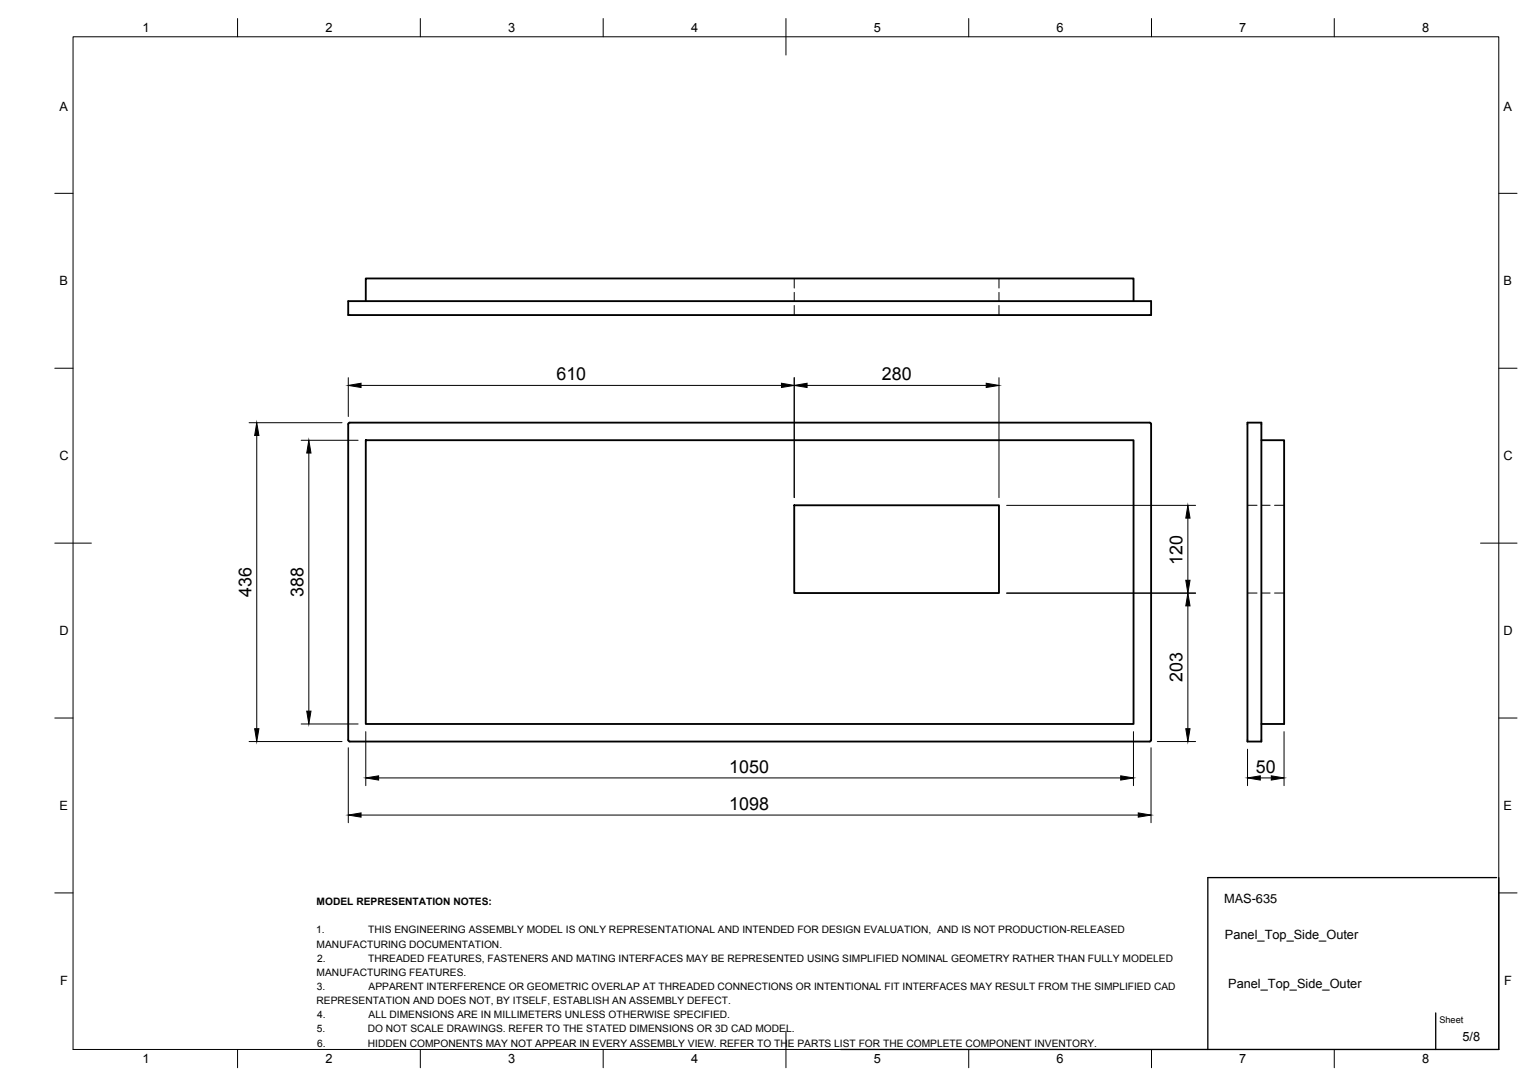
ISO-10303-21;
HEADER;
FILE_DESCRIPTION((''),'2;1');
FILE_NAME('Panel_Top_Side_Outer.step','2026-10-09T12:34:24-07:00',(''),(''),'','','');
FILE_SCHEMA (('AUTOMOTIVE_DESIGN { 1 0 10303 214 3 1 1 }'));
ENDSEC;
DATA;
#10=MECHANICAL_DESIGN_GEOMETRIC_PRESENTATION_REPRESENTATION('',(#61),#3759);
#49=SHAPE_REPRESENTATION_RELATIONSHIP('SRR','None',#3790,#55) ;
#55=ADVANCED_BREP_SHAPE_REPRESENTATION('',(#67),#3755) ;
#61=STYLED_ITEM('',(#3827),#67) ;
#67=MANIFOLD_SOLID_BREP('Body1',#2265) ;
#79=CYLINDRICAL_SURFACE('',#2421,0.2) ;
#80=CYLINDRICAL_SURFACE('',#2422,0.2) ;
#81=CYLINDRICAL_SURFACE('',#2423,0.2) ;
#82=CYLINDRICAL_SURFACE('',#2424,0.2) ;
#103=CIRCLE('',#2412,0.2) ;
#104=CIRCLE('',#2413,0.2) ;
#105=CIRCLE('',#2414,0.2) ;
#106=CIRCLE('',#2415,0.2) ;
#107=CIRCLE('',#2417,0.2) ;
#108=CIRCLE('',#2418,0.2) ;
#109=CIRCLE('',#2419,0.2) ;
#110=CIRCLE('',#2420,0.2) ;
#129=FACE_BOUND('',#322,.T.) ;
#130=FACE_BOUND('',#328,.T.) ;
#131=FACE_BOUND('',#330,.T.) ;
#187=FACE_OUTER_BOUND('',#317,.T.) ;
#188=FACE_OUTER_BOUND('',#318,.T.) ;
#189=FACE_OUTER_BOUND('',#319,.T.) ;
#190=FACE_OUTER_BOUND('',#320,.T.) ;
#191=FACE_OUTER_BOUND('',#321,.T.) ;
#192=FACE_OUTER_BOUND('',#323,.T.) ;
#193=FACE_OUTER_BOUND('',#324,.T.) ;
#194=FACE_OUTER_BOUND('',#325,.T.) ;
#195=FACE_OUTER_BOUND('',#326,.T.) ;
#196=FACE_OUTER_BOUND('',#327,.T.) ;
#197=FACE_OUTER_BOUND('',#329,.T.) ;
#198=FACE_OUTER_BOUND('',#331,.T.) ;
#199=FACE_OUTER_BOUND('',#332,.T.) ;
#200=FACE_OUTER_BOUND('',#333,.T.) ;
#201=FACE_OUTER_BOUND('',#334,.T.) ;
#202=FACE_OUTER_BOUND('',#335,.T.) ;
#203=FACE_OUTER_BOUND('',#336,.T.) ;
#204=FACE_OUTER_BOUND('',#337,.T.) ;
#205=FACE_OUTER_BOUND('',#338,.T.) ;
#317=EDGE_LOOP('',(#1679,#1680,#1681,#1682)) ;
#318=EDGE_LOOP('',(#1683,#1684,#1685,#1686)) ;
#319=EDGE_LOOP('',(#1687,#1688,#1689,#1690)) ;
#320=EDGE_LOOP('',(#1691,#1692,#1693,#1694)) ;
#321=EDGE_LOOP('',(#1695,#1696,#1697,#1698)) ;
#322=EDGE_LOOP('',(#1699,#1700,#1701,#1702)) ;
#323=EDGE_LOOP('',(#1703,#1704,#1705,#1706)) ;
#324=EDGE_LOOP('',(#1707,#1708,#1709,#1710)) ;
#325=EDGE_LOOP('',(#1711,#1712,#1713,#1714)) ;
#326=EDGE_LOOP('',(#1715,#1716,#1717,#1718)) ;
#327=EDGE_LOOP('',(#1719,#1720,#1721,#1722,#1723,#1724,#1725,#1726)) ;
#328=EDGE_LOOP('',(#1727,#1728,#1729,#1730)) ;
#329=EDGE_LOOP('',(#1731,#1732,#1733,#1734,#1735,#1736,#1737,#1738)) ;
#330=EDGE_LOOP('',(#1739,#1740,#1741,#1742)) ;
#331=EDGE_LOOP('',(#1743,#1744,#1745,#1746)) ;
#332=EDGE_LOOP('',(#1747,#1748,#1749,#1750)) ;
#333=EDGE_LOOP('',(#1751,#1752,#1753,#1754)) ;
#334=EDGE_LOOP('',(#1755,#1756,#1757,#1758)) ;
#335=EDGE_LOOP('',(#1759,#1760,#1761,#1762)) ;
#336=EDGE_LOOP('',(#1763,#1764,#1765,#1766)) ;
#337=EDGE_LOOP('',(#1767,#1768,#1769,#1770)) ;
#338=EDGE_LOOP('',(#1771,#1772,#1773,#1774)) ;
#507=LINE('',#3361,#775) ;
#508=LINE('',#3363,#776) ;
#509=LINE('',#3365,#777) ;
#510=LINE('',#3366,#778) ;
#511=LINE('',#3369,#779) ;
#512=LINE('',#3371,#780) ;
#513=LINE('',#3372,#781) ;
#514=LINE('',#3375,#782) ;
#515=LINE('',#3377,#783) ;
#516=LINE('',#3378,#784) ;
#517=LINE('',#3380,#785) ;
#518=LINE('',#3381,#786) ;
#519=LINE('',#3385,#787) ;
#520=LINE('',#3387,#788) ;
#521=LINE('',#3389,#789) ;
#522=LINE('',#3390,#790) ;
#523=LINE('',#3394,#791) ;
#524=LINE('',#3396,#792) ;
#525=LINE('',#3398,#793) ;
#526=LINE('',#3399,#794) ;
#527=LINE('',#3403,#795) ;
#528=LINE('',#3405,#796) ;
#529=LINE('',#3407,#797) ;
#530=LINE('',#3408,#798) ;
#531=LINE('',#3412,#799) ;
#532=LINE('',#3414,#800) ;
#533=LINE('',#3416,#801) ;
#534=LINE('',#3417,#802) ;
#535=LINE('',#3421,#803) ;
#536=LINE('',#3423,#804) ;
#537=LINE('',#3425,#805) ;
#538=LINE('',#3426,#806) ;
#539=LINE('',#3439,#807) ;
#540=LINE('',#3441,#808) ;
#541=LINE('',#3443,#809) ;
#542=LINE('',#3444,#810) ;
#543=LINE('',#3450,#811) ;
#544=LINE('',#3451,#812) ;
#545=LINE('',#3453,#813) ;
#546=LINE('',#3455,#814) ;
#775=VECTOR('',#2742,100.) ;
#776=VECTOR('',#2743,100.) ;
#777=VECTOR('',#2744,100.) ;
#778=VECTOR('',#2745,100.) ;
#779=VECTOR('',#2748,100.) ;
#780=VECTOR('',#2749,100.) ;
#781=VECTOR('',#2750,100.) ;
#782=VECTOR('',#2753,100.) ;
#783=VECTOR('',#2754,100.) ;
#784=VECTOR('',#2755,100.) ;
#785=VECTOR('',#2758,100.) ;
#786=VECTOR('',#2759,100.) ;
#787=VECTOR('',#2762,100.) ;
#788=VECTOR('',#2763,100.) ;
#789=VECTOR('',#2764,100.) ;
#790=VECTOR('',#2765,100.) ;
#791=VECTOR('',#2768,100.) ;
#792=VECTOR('',#2769,100.) ;
#793=VECTOR('',#2770,100.) ;
#794=VECTOR('',#2771,100.) ;
#795=VECTOR('',#2774,100.) ;
#796=VECTOR('',#2775,100.) ;
#797=VECTOR('',#2776,100.) ;
#798=VECTOR('',#2777,100.) ;
#799=VECTOR('',#2780,100.) ;
#800=VECTOR('',#2781,100.) ;
#801=VECTOR('',#2782,100.) ;
#802=VECTOR('',#2783,100.) ;
#803=VECTOR('',#2786,100.) ;
#804=VECTOR('',#2787,100.) ;
#805=VECTOR('',#2788,100.) ;
#806=VECTOR('',#2789,100.) ;
#807=VECTOR('',#2810,100.) ;
#808=VECTOR('',#2811,100.) ;
#809=VECTOR('',#2812,100.) ;
#810=VECTOR('',#2813,100.) ;
#811=VECTOR('',#2824,100.) ;
#812=VECTOR('',#2825,100.) ;
#813=VECTOR('',#2828,100.) ;
#814=VECTOR('',#2831,100.) ;
#1019=VERTEX_POINT('',#3359) ;
#1020=VERTEX_POINT('',#3360) ;
#1021=VERTEX_POINT('',#3362) ;
#1022=VERTEX_POINT('',#3364) ;
#1023=VERTEX_POINT('',#3368) ;
#1024=VERTEX_POINT('',#3370) ;
#1025=VERTEX_POINT('',#3374) ;
#1026=VERTEX_POINT('',#3376) ;
#1027=VERTEX_POINT('',#3383) ;
#1028=VERTEX_POINT('',#3384) ;
#1029=VERTEX_POINT('',#3386) ;
#1030=VERTEX_POINT('',#3388) ;
#1031=VERTEX_POINT('',#3392) ;
#1032=VERTEX_POINT('',#3393) ;
#1033=VERTEX_POINT('',#3395) ;
#1034=VERTEX_POINT('',#3397) ;
#1035=VERTEX_POINT('',#3401) ;
#1036=VERTEX_POINT('',#3402) ;
#1037=VERTEX_POINT('',#3404) ;
#1038=VERTEX_POINT('',#3406) ;
#1039=VERTEX_POINT('',#3410) ;
#1040=VERTEX_POINT('',#3411) ;
#1041=VERTEX_POINT('',#3413) ;
#1042=VERTEX_POINT('',#3415) ;
#1043=VERTEX_POINT('',#3419) ;
#1044=VERTEX_POINT('',#3420) ;
#1045=VERTEX_POINT('',#3422) ;
#1046=VERTEX_POINT('',#3424) ;
#1047=VERTEX_POINT('',#3437) ;
#1048=VERTEX_POINT('',#3438) ;
#1049=VERTEX_POINT('',#3440) ;
#1050=VERTEX_POINT('',#3442) ;
#1259=EDGE_CURVE('',#1019,#1020,#507,.T.) ;
#1260=EDGE_CURVE('',#1021,#1019,#508,.T.) ;
#1261=EDGE_CURVE('',#1021,#1022,#509,.T.) ;
#1262=EDGE_CURVE('',#1022,#1020,#510,.T.) ;
#1263=EDGE_CURVE('',#1019,#1023,#511,.T.) ;
#1264=EDGE_CURVE('',#1024,#1023,#512,.T.) ;
#1265=EDGE_CURVE('',#1021,#1024,#513,.T.) ;
#1266=EDGE_CURVE('',#1023,#1025,#514,.T.) ;
#1267=EDGE_CURVE('',#1026,#1025,#515,.T.) ;
#1268=EDGE_CURVE('',#1024,#1026,#516,.T.) ;
#1269=EDGE_CURVE('',#1020,#1025,#517,.T.) ;
#1270=EDGE_CURVE('',#1022,#1026,#518,.T.) ;
#1271=EDGE_CURVE('',#1027,#1028,#519,.T.) ;
#1272=EDGE_CURVE('',#1028,#1029,#520,.T.) ;
#1273=EDGE_CURVE('',#1029,#1030,#521,.T.) ;
#1274=EDGE_CURVE('',#1030,#1027,#522,.T.) ;
#1275=EDGE_CURVE('',#1031,#1032,#523,.T.) ;
#1276=EDGE_CURVE('',#1031,#1033,#524,.T.) ;
#1277=EDGE_CURVE('',#1033,#1034,#525,.T.) ;
#1278=EDGE_CURVE('',#1034,#1032,#526,.T.) ;
#1279=EDGE_CURVE('',#1035,#1036,#527,.T.) ;
#1280=EDGE_CURVE('',#1036,#1037,#528,.T.) ;
#1281=EDGE_CURVE('',#1038,#1037,#529,.T.) ;
#1282=EDGE_CURVE('',#1038,#1035,#530,.T.) ;
#1283=EDGE_CURVE('',#1039,#1040,#531,.T.) ;
#1284=EDGE_CURVE('',#1039,#1041,#532,.T.) ;
#1285=EDGE_CURVE('',#1041,#1042,#533,.T.) ;
#1286=EDGE_CURVE('',#1042,#1040,#534,.T.) ;
#1287=EDGE_CURVE('',#1043,#1044,#535,.T.) ;
#1288=EDGE_CURVE('',#1043,#1045,#536,.T.) ;
#1289=EDGE_CURVE('',#1045,#1046,#537,.T.) ;
#1290=EDGE_CURVE('',#1046,#1044,#538,.T.) ;
#1291=EDGE_CURVE('',#1045,#1031,#103,.T.) ;
#1292=EDGE_CURVE('',#1032,#1038,#104,.T.) ;
#1293=EDGE_CURVE('',#1037,#1042,#105,.T.) ;
#1294=EDGE_CURVE('',#1041,#1046,#106,.T.) ;
#1295=EDGE_CURVE('',#1033,#1043,#107,.T.) ;
#1296=EDGE_CURVE('',#1044,#1039,#108,.T.) ;
#1297=EDGE_CURVE('',#1040,#1036,#109,.T.) ;
#1298=EDGE_CURVE('',#1035,#1034,#110,.T.) ;
#1299=EDGE_CURVE('',#1047,#1048,#539,.T.) ;
#1300=EDGE_CURVE('',#1049,#1047,#540,.T.) ;
#1301=EDGE_CURVE('',#1050,#1049,#541,.T.) ;
#1302=EDGE_CURVE('',#1048,#1050,#542,.T.) ;
#1303=EDGE_CURVE('',#1028,#1047,#543,.T.) ;
#1304=EDGE_CURVE('',#1029,#1048,#544,.T.) ;
#1305=EDGE_CURVE('',#1027,#1049,#545,.T.) ;
#1306=EDGE_CURVE('',#1030,#1050,#546,.T.) ;
#1679=ORIENTED_EDGE('',*,*,#1259,.F.) ;
#1680=ORIENTED_EDGE('',*,*,#1260,.F.) ;
#1681=ORIENTED_EDGE('',*,*,#1261,.T.) ;
#1682=ORIENTED_EDGE('',*,*,#1262,.T.) ;
#1683=ORIENTED_EDGE('',*,*,#1260,.T.) ;
#1684=ORIENTED_EDGE('',*,*,#1263,.T.) ;
#1685=ORIENTED_EDGE('',*,*,#1264,.F.) ;
#1686=ORIENTED_EDGE('',*,*,#1265,.F.) ;
#1687=ORIENTED_EDGE('',*,*,#1264,.T.) ;
#1688=ORIENTED_EDGE('',*,*,#1266,.T.) ;
#1689=ORIENTED_EDGE('',*,*,#1267,.F.) ;
#1690=ORIENTED_EDGE('',*,*,#1268,.F.) ;
#1691=ORIENTED_EDGE('',*,*,#1269,.F.) ;
#1692=ORIENTED_EDGE('',*,*,#1262,.F.) ;
#1693=ORIENTED_EDGE('',*,*,#1270,.T.) ;
#1694=ORIENTED_EDGE('',*,*,#1267,.T.) ;
#1695=ORIENTED_EDGE('',*,*,#1261,.F.) ;
#1696=ORIENTED_EDGE('',*,*,#1265,.T.) ;
#1697=ORIENTED_EDGE('',*,*,#1268,.T.) ;
#1698=ORIENTED_EDGE('',*,*,#1270,.F.) ;
#1699=ORIENTED_EDGE('',*,*,#1271,.T.) ;
#1700=ORIENTED_EDGE('',*,*,#1272,.T.) ;
#1701=ORIENTED_EDGE('',*,*,#1273,.T.) ;
#1702=ORIENTED_EDGE('',*,*,#1274,.T.) ;
#1703=ORIENTED_EDGE('',*,*,#1275,.F.) ;
#1704=ORIENTED_EDGE('',*,*,#1276,.T.) ;
#1705=ORIENTED_EDGE('',*,*,#1277,.T.) ;
#1706=ORIENTED_EDGE('',*,*,#1278,.T.) ;
#1707=ORIENTED_EDGE('',*,*,#1279,.T.) ;
#1708=ORIENTED_EDGE('',*,*,#1280,.T.) ;
#1709=ORIENTED_EDGE('',*,*,#1281,.F.) ;
#1710=ORIENTED_EDGE('',*,*,#1282,.T.) ;
#1711=ORIENTED_EDGE('',*,*,#1283,.F.) ;
#1712=ORIENTED_EDGE('',*,*,#1284,.T.) ;
#1713=ORIENTED_EDGE('',*,*,#1285,.T.) ;
#1714=ORIENTED_EDGE('',*,*,#1286,.T.) ;
#1715=ORIENTED_EDGE('',*,*,#1287,.F.) ;
#1716=ORIENTED_EDGE('',*,*,#1288,.T.) ;
#1717=ORIENTED_EDGE('',*,*,#1289,.T.) ;
#1718=ORIENTED_EDGE('',*,*,#1290,.T.) ;
#1719=ORIENTED_EDGE('',*,*,#1289,.F.) ;
#1720=ORIENTED_EDGE('',*,*,#1291,.T.) ;
#1721=ORIENTED_EDGE('',*,*,#1275,.T.) ;
#1722=ORIENTED_EDGE('',*,*,#1292,.T.) ;
#1723=ORIENTED_EDGE('',*,*,#1281,.T.) ;
#1724=ORIENTED_EDGE('',*,*,#1293,.T.) ;
#1725=ORIENTED_EDGE('',*,*,#1285,.F.) ;
#1726=ORIENTED_EDGE('',*,*,#1294,.T.) ;
#1727=ORIENTED_EDGE('',*,*,#1263,.F.) ;
#1728=ORIENTED_EDGE('',*,*,#1259,.T.) ;
#1729=ORIENTED_EDGE('',*,*,#1269,.T.) ;
#1730=ORIENTED_EDGE('',*,*,#1266,.F.) ;
#1731=ORIENTED_EDGE('',*,*,#1277,.F.) ;
#1732=ORIENTED_EDGE('',*,*,#1295,.T.) ;
#1733=ORIENTED_EDGE('',*,*,#1287,.T.) ;
#1734=ORIENTED_EDGE('',*,*,#1296,.T.) ;
#1735=ORIENTED_EDGE('',*,*,#1283,.T.) ;
#1736=ORIENTED_EDGE('',*,*,#1297,.T.) ;
#1737=ORIENTED_EDGE('',*,*,#1279,.F.) ;
#1738=ORIENTED_EDGE('',*,*,#1298,.T.) ;
#1739=ORIENTED_EDGE('',*,*,#1299,.F.) ;
#1740=ORIENTED_EDGE('',*,*,#1300,.F.) ;
#1741=ORIENTED_EDGE('',*,*,#1301,.F.) ;
#1742=ORIENTED_EDGE('',*,*,#1302,.F.) ;
#1743=ORIENTED_EDGE('',*,*,#1291,.F.) ;
#1744=ORIENTED_EDGE('',*,*,#1288,.F.) ;
#1745=ORIENTED_EDGE('',*,*,#1295,.F.) ;
#1746=ORIENTED_EDGE('',*,*,#1276,.F.) ;
#1747=ORIENTED_EDGE('',*,*,#1294,.F.) ;
#1748=ORIENTED_EDGE('',*,*,#1284,.F.) ;
#1749=ORIENTED_EDGE('',*,*,#1296,.F.) ;
#1750=ORIENTED_EDGE('',*,*,#1290,.F.) ;
#1751=ORIENTED_EDGE('',*,*,#1293,.F.) ;
#1752=ORIENTED_EDGE('',*,*,#1280,.F.) ;
#1753=ORIENTED_EDGE('',*,*,#1297,.F.) ;
#1754=ORIENTED_EDGE('',*,*,#1286,.F.) ;
#1755=ORIENTED_EDGE('',*,*,#1292,.F.) ;
#1756=ORIENTED_EDGE('',*,*,#1278,.F.) ;
#1757=ORIENTED_EDGE('',*,*,#1298,.F.) ;
#1758=ORIENTED_EDGE('',*,*,#1282,.F.) ;
#1759=ORIENTED_EDGE('',*,*,#1303,.T.) ;
#1760=ORIENTED_EDGE('',*,*,#1299,.T.) ;
#1761=ORIENTED_EDGE('',*,*,#1304,.F.) ;
#1762=ORIENTED_EDGE('',*,*,#1272,.F.) ;
#1763=ORIENTED_EDGE('',*,*,#1305,.T.) ;
#1764=ORIENTED_EDGE('',*,*,#1300,.T.) ;
#1765=ORIENTED_EDGE('',*,*,#1303,.F.) ;
#1766=ORIENTED_EDGE('',*,*,#1271,.F.) ;
#1767=ORIENTED_EDGE('',*,*,#1306,.T.) ;
#1768=ORIENTED_EDGE('',*,*,#1301,.T.) ;
#1769=ORIENTED_EDGE('',*,*,#1305,.F.) ;
#1770=ORIENTED_EDGE('',*,*,#1274,.F.) ;
#1771=ORIENTED_EDGE('',*,*,#1304,.T.) ;
#1772=ORIENTED_EDGE('',*,*,#1302,.T.) ;
#1773=ORIENTED_EDGE('',*,*,#1306,.F.) ;
#1774=ORIENTED_EDGE('',*,*,#1273,.F.) ;
#2077=PLANE('',#2402) ;
#2078=PLANE('',#2403) ;
#2079=PLANE('',#2404) ;
#2080=PLANE('',#2405) ;
#2081=PLANE('',#2406) ;
#2082=PLANE('',#2407) ;
#2083=PLANE('',#2408) ;
#2084=PLANE('',#2409) ;
#2085=PLANE('',#2410) ;
#2086=PLANE('',#2411) ;
#2087=PLANE('',#2416) ;
#2088=PLANE('',#2425) ;
#2089=PLANE('',#2426) ;
#2090=PLANE('',#2427) ;
#2091=PLANE('',#2428) ;
#2189=ADVANCED_FACE('',(#187),#2077,.T.) ;
#2190=ADVANCED_FACE('',(#188),#2078,.F.) ;
#2191=ADVANCED_FACE('',(#189),#2079,.F.) ;
#2192=ADVANCED_FACE('',(#190),#2080,.T.) ;
#2193=ADVANCED_FACE('',(#191,#129),#2081,.F.) ;
#2194=ADVANCED_FACE('',(#192),#2082,.F.) ;
#2195=ADVANCED_FACE('',(#193),#2083,.F.) ;
#2196=ADVANCED_FACE('',(#194),#2084,.T.) ;
#2197=ADVANCED_FACE('',(#195),#2085,.T.) ;
#2198=ADVANCED_FACE('',(#196,#130),#2086,.T.) ;
#2199=ADVANCED_FACE('',(#197,#131),#2087,.T.) ;
#2200=ADVANCED_FACE('',(#198),#79,.T.) ;
#2201=ADVANCED_FACE('',(#199),#80,.T.) ;
#2202=ADVANCED_FACE('',(#200),#81,.T.) ;
#2203=ADVANCED_FACE('',(#201),#82,.T.) ;
#2204=ADVANCED_FACE('',(#202),#2088,.F.) ;
#2205=ADVANCED_FACE('',(#203),#2089,.F.) ;
#2206=ADVANCED_FACE('',(#204),#2090,.F.) ;
#2207=ADVANCED_FACE('',(#205),#2091,.F.) ;
#2265=CLOSED_SHELL('',(#2189,#2190,#2191,#2192,#2193,#2194,#2195,#2196,
#2197,#2198,#2199,#2200,#2201,#2202,#2203,#2204,#2205,#2206,#2207)) ;
#2401=AXIS2_PLACEMENT_3D('',#3357,#2738,#2739) ;
#2402=AXIS2_PLACEMENT_3D('',#3358,#2740,#2741) ;
#2403=AXIS2_PLACEMENT_3D('',#3367,#2746,#2747) ;
#2404=AXIS2_PLACEMENT_3D('',#3373,#2751,#2752) ;
#2405=AXIS2_PLACEMENT_3D('',#3379,#2756,#2757) ;
#2406=AXIS2_PLACEMENT_3D('',#3382,#2760,#2761) ;
#2407=AXIS2_PLACEMENT_3D('',#3391,#2766,#2767) ;
#2408=AXIS2_PLACEMENT_3D('',#3400,#2772,#2773) ;
#2409=AXIS2_PLACEMENT_3D('',#3409,#2778,#2779) ;
#2410=AXIS2_PLACEMENT_3D('',#3418,#2784,#2785) ;
#2411=AXIS2_PLACEMENT_3D('',#3427,#2790,#2791) ;
#2412=AXIS2_PLACEMENT_3D('',#3428,#2792,#2793) ;
#2413=AXIS2_PLACEMENT_3D('',#3429,#2794,#2795) ;
#2414=AXIS2_PLACEMENT_3D('',#3430,#2796,#2797) ;
#2415=AXIS2_PLACEMENT_3D('',#3431,#2798,#2799) ;
#2416=AXIS2_PLACEMENT_3D('',#3432,#2800,#2801) ;
#2417=AXIS2_PLACEMENT_3D('',#3433,#2802,#2803) ;
#2418=AXIS2_PLACEMENT_3D('',#3434,#2804,#2805) ;
#2419=AXIS2_PLACEMENT_3D('',#3435,#2806,#2807) ;
#2420=AXIS2_PLACEMENT_3D('',#3436,#2808,#2809) ;
#2421=AXIS2_PLACEMENT_3D('',#3445,#2814,#2815) ;
#2422=AXIS2_PLACEMENT_3D('',#3446,#2816,#2817) ;
#2423=AXIS2_PLACEMENT_3D('',#3447,#2818,#2819) ;
#2424=AXIS2_PLACEMENT_3D('',#3448,#2820,#2821) ;
#2425=AXIS2_PLACEMENT_3D('',#3449,#2822,#2823) ;
#2426=AXIS2_PLACEMENT_3D('',#3452,#2826,#2827) ;
#2427=AXIS2_PLACEMENT_3D('',#3454,#2829,#2830) ;
#2428=AXIS2_PLACEMENT_3D('',#3456,#2832,#2833) ;
#2738=DIRECTION('axis',(0.,0.,1.)) ;
#2739=DIRECTION('refdir',(1.,0.,0.)) ;
#2740=DIRECTION('center_axis',(1.58603289232165E-16,-1.,0.)) ;
#2741=DIRECTION('ref_axis',(1.,1.58603289232165E-16,0.)) ;
#2742=DIRECTION('',(-1.,-1.58603289232165E-16,0.)) ;
#2743=DIRECTION('',(0.,0.,-1.)) ;
#2744=DIRECTION('',(-1.,-1.58603289232165E-16,0.)) ;
#2745=DIRECTION('',(0.,0.,-1.)) ;
#2746=DIRECTION('center_axis',(-1.,0.,0.)) ;
#2747=DIRECTION('ref_axis',(0.,0.,1.)) ;
#2748=DIRECTION('',(0.,1.,0.)) ;
#2749=DIRECTION('',(0.,0.,-1.)) ;
#2750=DIRECTION('',(0.,1.,0.)) ;
#2751=DIRECTION('center_axis',(1.05735526154777E-16,-1.,0.)) ;
#2752=DIRECTION('ref_axis',(1.,1.05735526154777E-16,0.)) ;
#2753=DIRECTION('',(-1.,-1.05735526154777E-16,0.)) ;
#2754=DIRECTION('',(0.,0.,-1.)) ;
#2755=DIRECTION('',(-1.,-1.05735526154777E-16,0.)) ;
#2756=DIRECTION('center_axis',(-1.,0.,0.)) ;
#2757=DIRECTION('ref_axis',(0.,0.,1.)) ;
#2758=DIRECTION('',(0.,1.,0.)) ;
#2759=DIRECTION('',(0.,1.,0.)) ;
#2760=DIRECTION('center_axis',(0.,0.,-1.)) ;
#2761=DIRECTION('ref_axis',(-1.,0.,0.)) ;
#2762=DIRECTION('',(1.,-9.91270557701033E-17,0.)) ;
#2763=DIRECTION('',(0.,-1.,0.)) ;
#2764=DIRECTION('',(-1.,1.48690583655155E-16,0.)) ;
#2765=DIRECTION('',(0.,1.,0.)) ;
#2766=DIRECTION('center_axis',(-1.,0.,0.)) ;
#2767=DIRECTION('ref_axis',(0.,0.,1.)) ;
#2768=DIRECTION('',(0.,1.,0.)) ;
#2769=DIRECTION('',(0.,0.,-1.)) ;
#2770=DIRECTION('',(0.,1.,0.)) ;
#2771=DIRECTION('',(0.,0.,1.)) ;
#2772=DIRECTION('center_axis',(1.26391510089385E-16,-1.,0.)) ;
#2773=DIRECTION('ref_axis',(1.,1.26391510089385E-16,0.)) ;
#2774=DIRECTION('',(-1.,-1.26391510089385E-16,0.)) ;
#2775=DIRECTION('',(0.,0.,1.)) ;
#2776=DIRECTION('',(-1.,-1.26391510089385E-16,0.)) ;
#2777=DIRECTION('',(0.,0.,-1.)) ;
#2778=DIRECTION('center_axis',(-1.,0.,0.)) ;
#2779=DIRECTION('ref_axis',(0.,0.,1.)) ;
#2780=DIRECTION('',(0.,1.,0.)) ;
#2781=DIRECTION('',(0.,0.,1.)) ;
#2782=DIRECTION('',(0.,1.,0.)) ;
#2783=DIRECTION('',(0.,0.,-1.)) ;
#2784=DIRECTION('center_axis',(1.51669812107262E-16,-1.,0.)) ;
#2785=DIRECTION('ref_axis',(1.,1.51669812107262E-16,0.)) ;
#2786=DIRECTION('',(-1.,-1.51669812107262E-16,0.)) ;
#2787=DIRECTION('',(0.,0.,1.)) ;
#2788=DIRECTION('',(-1.,-1.51669812107262E-16,0.)) ;
#2789=DIRECTION('',(0.,0.,-1.)) ;
#2790=DIRECTION('center_axis',(0.,0.,1.)) ;
#2791=DIRECTION('ref_axis',(1.,0.,0.)) ;
#2792=DIRECTION('center_axis',(0.,0.,1.)) ;
#2793=DIRECTION('ref_axis',(1.,0.,0.)) ;
#2794=DIRECTION('center_axis',(0.,0.,1.)) ;
#2795=DIRECTION('ref_axis',(1.,0.,0.)) ;
#2796=DIRECTION('center_axis',(0.,0.,1.)) ;
#2797=DIRECTION('ref_axis',(1.,0.,0.)) ;
#2798=DIRECTION('center_axis',(0.,0.,1.)) ;
#2799=DIRECTION('ref_axis',(1.,0.,0.)) ;
#2800=DIRECTION('center_axis',(0.,0.,-1.)) ;
#2801=DIRECTION('ref_axis',(-1.,0.,0.)) ;
#2802=DIRECTION('center_axis',(0.,0.,-1.)) ;
#2803=DIRECTION('ref_axis',(-1.,0.,0.)) ;
#2804=DIRECTION('center_axis',(0.,0.,-1.)) ;
#2805=DIRECTION('ref_axis',(-1.,0.,0.)) ;
#2806=DIRECTION('center_axis',(0.,0.,-1.)) ;
#2807=DIRECTION('ref_axis',(-1.,0.,0.)) ;
#2808=DIRECTION('center_axis',(0.,0.,-1.)) ;
#2809=DIRECTION('ref_axis',(-1.,0.,0.)) ;
#2810=DIRECTION('',(0.,-1.,0.)) ;
#2811=DIRECTION('',(1.,-9.91270557701033E-17,0.)) ;
#2812=DIRECTION('',(0.,1.,0.)) ;
#2813=DIRECTION('',(-1.,1.48690583655155E-16,0.)) ;
#2814=DIRECTION('center_axis',(0.,0.,1.)) ;
#2815=DIRECTION('ref_axis',(1.,0.,0.)) ;
#2816=DIRECTION('center_axis',(0.,0.,-1.)) ;
#2817=DIRECTION('ref_axis',(-1.,0.,0.)) ;
#2818=DIRECTION('center_axis',(0.,0.,1.)) ;
#2819=DIRECTION('ref_axis',(1.,0.,0.)) ;
#2820=DIRECTION('center_axis',(0.,0.,-1.)) ;
#2821=DIRECTION('ref_axis',(-1.,0.,0.)) ;
#2822=DIRECTION('center_axis',(1.,0.,0.)) ;
#2823=DIRECTION('ref_axis',(0.,0.,-1.)) ;
#2824=DIRECTION('',(0.,0.,-1.)) ;
#2825=DIRECTION('',(0.,0.,-1.)) ;
#2826=DIRECTION('center_axis',(9.91270557701033E-17,1.,0.)) ;
#2827=DIRECTION('ref_axis',(-1.,9.91270557701033E-17,0.)) ;
#2828=DIRECTION('',(0.,0.,-1.)) ;
#2829=DIRECTION('center_axis',(-1.,0.,0.)) ;
#2830=DIRECTION('ref_axis',(0.,0.,1.)) ;
#2831=DIRECTION('',(0.,0.,-1.)) ;
#2832=DIRECTION('center_axis',(-1.48690583655155E-16,-1.,0.)) ;
#2833=DIRECTION('ref_axis',(1.,-1.48690583655155E-16,0.)) ;
#3357=CARTESIAN_POINT('',(0.,0.,0.)) ;
#3358=CARTESIAN_POINT('Origin',(52.5,-19.4,5.)) ;
#3359=CARTESIAN_POINT('',(52.5,-19.4,1.9)) ;
#3360=CARTESIAN_POINT('',(-52.5,-19.4,1.9)) ;
#3361=CARTESIAN_POINT('',(52.5,-19.4,1.9)) ;
#3362=CARTESIAN_POINT('',(52.5,-19.4,5.)) ;
#3363=CARTESIAN_POINT('',(52.5,-19.4,5.)) ;
#3364=CARTESIAN_POINT('',(-52.5,-19.4,5.)) ;
#3365=CARTESIAN_POINT('',(52.5,-19.4,5.)) ;
#3366=CARTESIAN_POINT('',(-52.5,-19.4,5.)) ;
#3367=CARTESIAN_POINT('Origin',(52.5,-19.4,5.)) ;
#3368=CARTESIAN_POINT('',(52.5,19.4,1.9)) ;
#3369=CARTESIAN_POINT('',(52.5,-19.4,1.9)) ;
#3370=CARTESIAN_POINT('',(52.5,19.4,5.)) ;
#3371=CARTESIAN_POINT('',(52.5,19.4,5.)) ;
#3372=CARTESIAN_POINT('',(52.5,-19.4,5.)) ;
#3373=CARTESIAN_POINT('Origin',(52.5,19.4,5.)) ;
#3374=CARTESIAN_POINT('',(-52.5,19.4,1.9)) ;
#3375=CARTESIAN_POINT('',(52.5,19.4,1.9)) ;
#3376=CARTESIAN_POINT('',(-52.5,19.4,5.)) ;
#3377=CARTESIAN_POINT('',(-52.5,19.4,5.)) ;
#3378=CARTESIAN_POINT('',(52.5,19.4,5.)) ;
#3379=CARTESIAN_POINT('Origin',(-52.5,-19.4,5.)) ;
#3380=CARTESIAN_POINT('',(-52.5,-19.4,1.9)) ;
#3381=CARTESIAN_POINT('',(-52.5,-19.4,5.)) ;
#3382=CARTESIAN_POINT('Origin',(0.,0.,5.)) ;
#3383=CARTESIAN_POINT('',(6.1,10.5,5.)) ;
#3384=CARTESIAN_POINT('',(34.1,10.5,5.)) ;
#3385=CARTESIAN_POINT('',(1.04083408558609E-15,10.5,5.)) ;
#3386=CARTESIAN_POINT('',(34.1,-1.5,5.)) ;
#3387=CARTESIAN_POINT('',(34.1,0.,5.)) ;
#3388=CARTESIAN_POINT('',(6.1,-1.49999999999999,5.)) ;
#3389=CARTESIAN_POINT('',(-2.23035875482731E-16,-1.49999999999999,5.)) ;
#3390=CARTESIAN_POINT('',(6.1,0.,5.)) ;
#3391=CARTESIAN_POINT('Origin',(54.9,-21.8,1.9)) ;
#3392=CARTESIAN_POINT('',(54.9,-21.6,1.9)) ;
#3393=CARTESIAN_POINT('',(54.9,21.6,1.9)) ;
#3394=CARTESIAN_POINT('',(54.9,-21.8,1.9)) ;
#3395=CARTESIAN_POINT('',(54.9,-21.6,0.)) ;
#3396=CARTESIAN_POINT('',(54.9,-21.6,0.)) ;
#3397=CARTESIAN_POINT('',(54.9,21.6,0.)) ;
#3398=CARTESIAN_POINT('',(54.9,-21.8,0.)) ;
#3399=CARTESIAN_POINT('',(54.9,21.6,1.9)) ;
#3400=CARTESIAN_POINT('Origin',(54.9,21.8,1.9)) ;
#3401=CARTESIAN_POINT('',(54.7,21.8,0.)) ;
#3402=CARTESIAN_POINT('',(-54.7,21.8,0.)) ;
#3403=CARTESIAN_POINT('',(54.9,21.8,0.)) ;
#3404=CARTESIAN_POINT('',(-54.7,21.8,1.9)) ;
#3405=CARTESIAN_POINT('',(-54.7,21.8,1.9)) ;
#3406=CARTESIAN_POINT('',(54.7,21.8,1.9)) ;
#3407=CARTESIAN_POINT('',(54.9,21.8,1.9)) ;
#3408=CARTESIAN_POINT('',(54.7,21.8,1.9)) ;
#3409=CARTESIAN_POINT('Origin',(-54.9,-21.8,1.9)) ;
#3410=CARTESIAN_POINT('',(-54.9,-21.6,0.)) ;
#3411=CARTESIAN_POINT('',(-54.9,21.6,0.)) ;
#3412=CARTESIAN_POINT('',(-54.9,-21.8,0.)) ;
#3413=CARTESIAN_POINT('',(-54.9,-21.6,1.9)) ;
#3414=CARTESIAN_POINT('',(-54.9,-21.6,1.9)) ;
#3415=CARTESIAN_POINT('',(-54.9,21.6,1.9)) ;
#3416=CARTESIAN_POINT('',(-54.9,-21.8,1.9)) ;
#3417=CARTESIAN_POINT('',(-54.9,21.6,0.)) ;
#3418=CARTESIAN_POINT('Origin',(54.9,-21.8,1.9)) ;
#3419=CARTESIAN_POINT('',(54.7,-21.8,0.)) ;
#3420=CARTESIAN_POINT('',(-54.7,-21.8,0.)) ;
#3421=CARTESIAN_POINT('',(54.9,-21.8,0.)) ;
#3422=CARTESIAN_POINT('',(54.7,-21.8,1.9)) ;
#3423=CARTESIAN_POINT('',(54.7,-21.8,1.9)) ;
#3424=CARTESIAN_POINT('',(-54.7,-21.8,1.9)) ;
#3425=CARTESIAN_POINT('',(54.9,-21.8,1.9)) ;
#3426=CARTESIAN_POINT('',(-54.7,-21.8,1.9)) ;
#3427=CARTESIAN_POINT('Origin',(0.,0.,1.9)) ;
#3428=CARTESIAN_POINT('Origin',(54.7,-21.6,1.9)) ;
#3429=CARTESIAN_POINT('Origin',(54.7,21.6,1.9)) ;
#3430=CARTESIAN_POINT('Origin',(-54.7,21.6,1.9)) ;
#3431=CARTESIAN_POINT('Origin',(-54.7,-21.6,1.9)) ;
#3432=CARTESIAN_POINT('Origin',(0.,0.,0.)) ;
#3433=CARTESIAN_POINT('Origin',(54.7,-21.6,0.)) ;
#3434=CARTESIAN_POINT('Origin',(-54.7,-21.6,0.)) ;
#3435=CARTESIAN_POINT('Origin',(-54.7,21.6,0.)) ;
#3436=CARTESIAN_POINT('Origin',(54.7,21.6,0.)) ;
#3437=CARTESIAN_POINT('',(34.1,10.5,0.)) ;
#3438=CARTESIAN_POINT('',(34.1,-1.5,0.)) ;
#3439=CARTESIAN_POINT('',(34.1,-1.5,0.)) ;
#3440=CARTESIAN_POINT('',(6.1,10.5,0.)) ;
#3441=CARTESIAN_POINT('',(6.1,10.5,0.)) ;
#3442=CARTESIAN_POINT('',(6.1,-1.49999999999999,0.)) ;
#3443=CARTESIAN_POINT('',(6.1,-1.49999999999999,0.)) ;
#3444=CARTESIAN_POINT('',(6.1,-1.49999999999999,0.)) ;
#3445=CARTESIAN_POINT('Origin',(54.7,-21.6,1.9)) ;
#3446=CARTESIAN_POINT('Origin',(-54.7,-21.6,1.9)) ;
#3447=CARTESIAN_POINT('Origin',(-54.7,21.6,1.9)) ;
#3448=CARTESIAN_POINT('Origin',(54.7,21.6,1.9)) ;
#3449=CARTESIAN_POINT('Origin',(34.1,-1.5,6.)) ;
#3450=CARTESIAN_POINT('',(34.1,10.5,6.)) ;
#3451=CARTESIAN_POINT('',(34.1,-1.5,6.)) ;
#3452=CARTESIAN_POINT('Origin',(6.1,10.5,6.)) ;
#3453=CARTESIAN_POINT('',(6.1,10.5,6.)) ;
#3454=CARTESIAN_POINT('Origin',(6.1,-1.49999999999999,6.)) ;
#3455=CARTESIAN_POINT('',(6.1,-1.49999999999999,6.)) ;
#3456=CARTESIAN_POINT('Origin',(6.1,-1.49999999999999,6.)) ;
#3747=UNCERTAINTY_MEASURE_WITH_UNIT(LENGTH_MEASURE(0.001),#3760,
'DISTANCE_ACCURACY_VALUE',
'Maximum model space distance between geometric entities at asserted c
onnectivities') ;
#3751=UNCERTAINTY_MEASURE_WITH_UNIT(LENGTH_MEASURE(0.001),#3760,
'DISTANCE_ACCURACY_VALUE',
'Maximum model space distance between geometric entities at asserted c
onnectivities') ;
#3755=(
GEOMETRIC_REPRESENTATION_CONTEXT(3)
GLOBAL_UNCERTAINTY_ASSIGNED_CONTEXT((#3747))
GLOBAL_UNIT_ASSIGNED_CONTEXT((#3760,#3762,#3763))
REPRESENTATION_CONTEXT('','3D')
) ;
#3759=(
GEOMETRIC_REPRESENTATION_CONTEXT(3)
GLOBAL_UNCERTAINTY_ASSIGNED_CONTEXT((#3751))
GLOBAL_UNIT_ASSIGNED_CONTEXT((#3760,#3762,#3763))
REPRESENTATION_CONTEXT('','3D')
) ;
#3760=(
LENGTH_UNIT()
NAMED_UNIT(*)
SI_UNIT(.CENTI.,.METRE.)
) ;
#3762=(
NAMED_UNIT(*)
PLANE_ANGLE_UNIT()
SI_UNIT($,.RADIAN.)
) ;
#3763=(
NAMED_UNIT(*)
SI_UNIT($,.STERADIAN.)
SOLID_ANGLE_UNIT()
) ;
#3767=SHAPE_DEFINITION_REPRESENTATION(#3774,#3790) ;
#3774=PRODUCT_DEFINITION_SHAPE('',$,#3798) ;
#3790=SHAPE_REPRESENTATION('',(#2401),#3755) ;
#3794=PRODUCT_DEFINITION_CONTEXT('part definition',#3817,'design') ;
#3798=PRODUCT_DEFINITION('Panel_Top_Side_Outer',
'Panel_Top_Side_Outer',#3805,#3794) ;
#3805=PRODUCT_DEFINITION_FORMATION('',$,#3822) ;
#3817=APPLICATION_CONTEXT(
'Core Data for Automotive Mechanical Design Process') ;
#3818=PRODUCT_CONTEXT('part definition',#3817,'mechanical') ;
#3822=PRODUCT('Panel_Top_Side_Outer','Panel_Top_Side_Outer',$,(#3818)) ;
#3827=PRESENTATION_STYLE_ASSIGNMENT((#3829)) ;
#3829=SURFACE_STYLE_USAGE(.BOTH.,#3831) ;
#3831=SURFACE_SIDE_STYLE('',(#3833)) ;
#3833=SURFACE_STYLE_FILL_AREA(#3835) ;
#3835=FILL_AREA_STYLE('Opaque(179,179,179)',(#3837)) ;
#3837=FILL_AREA_STYLE_COLOUR('Opaque(179,179,179)',#3839) ;
#3839=COLOUR_RGB('Opaque(179,179,179)', 0.09019608, 0.27058824, 0.51372549) ;
ENDSEC;
END-ISO-10303-21;
